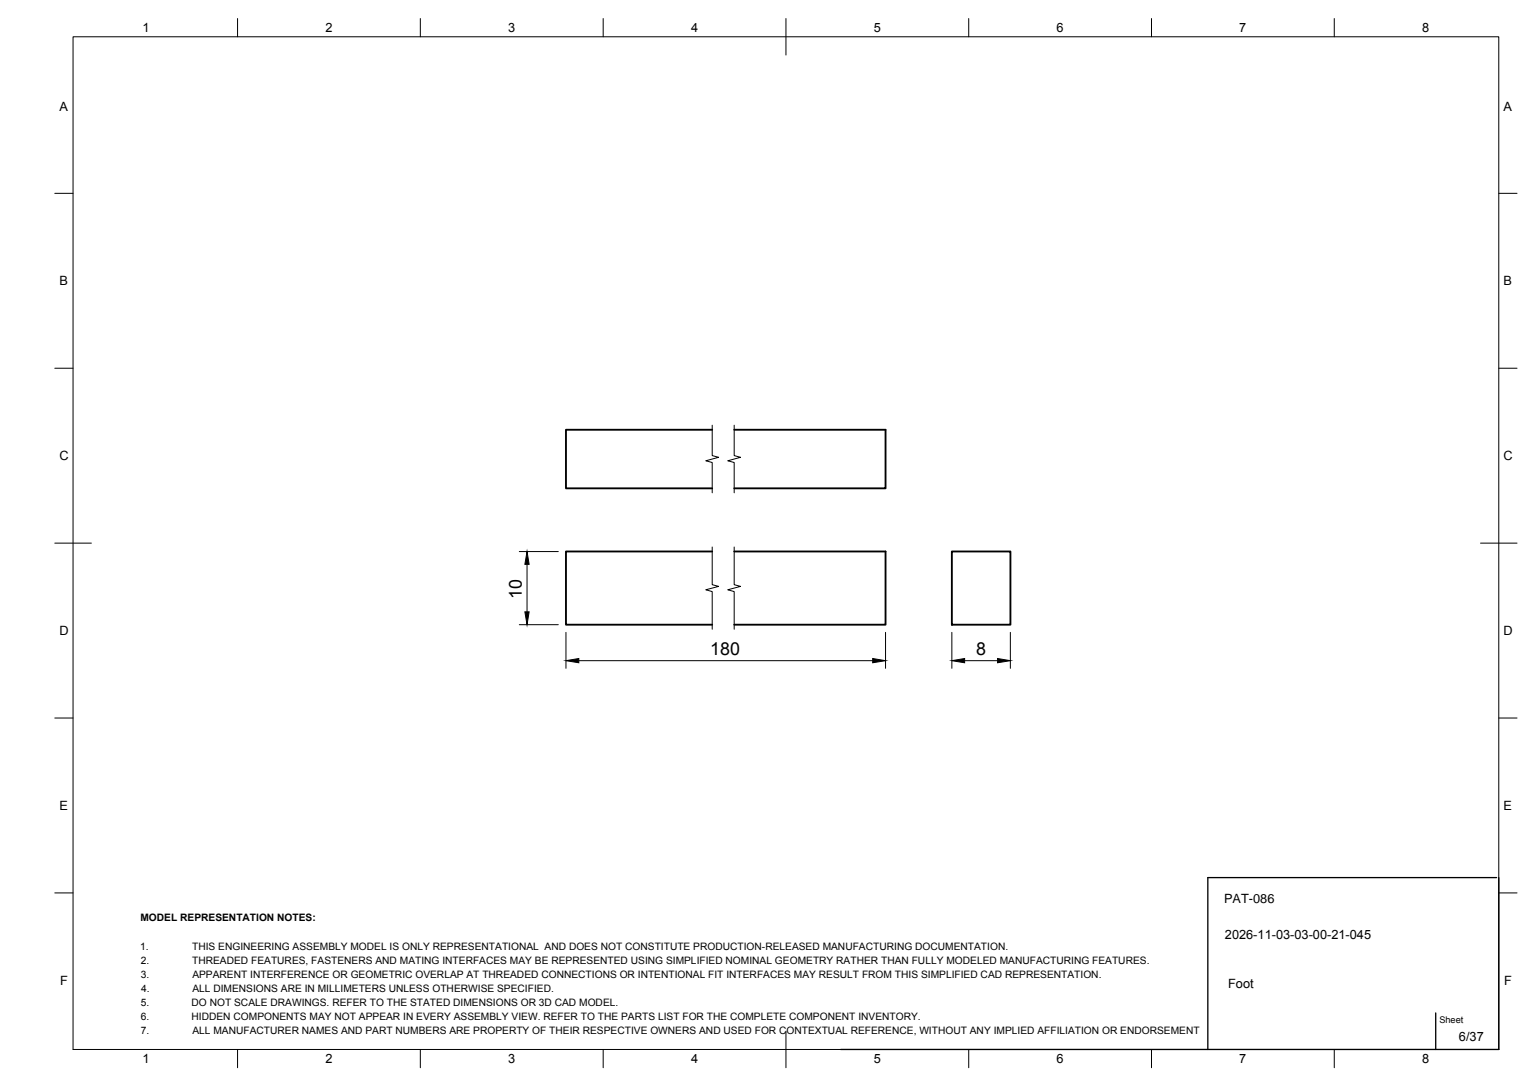
ISO-10303-21;
HEADER;
/* Generated by software containing ST-Developer
 * from STEP Tools, Inc. (www.steptools.com) 
 */

FILE_DESCRIPTION(
/* description */ ('Ratchet and pawl hand winch drum'),
/* implementation_level */ '2;1');

FILE_NAME(
/* name */ 'Foot.step',
/* time_stamp */ '2026-10-27T12:42:58-07:00',
/* author */ (''),
/* organization */ (''),
/* preprocessor_version */ 'ST-DEVELOPER v20.2',
/* originating_system */ 'Autodesk Translation Framework v15.17.0.0',
/* authorisation */ '');

FILE_SCHEMA (('AUTOMOTIVE_DESIGN { 1 0 10303 214 3 1 1 }'));
ENDSEC;

DATA;
#10=MECHANICAL_DESIGN_GEOMETRIC_PRESENTATION_REPRESENTATION('',(#390),#11801);
#322=SHAPE_REPRESENTATION_RELATIONSHIP('SRR','None',#11948,#356);
#356=ADVANCED_BREP_SHAPE_REPRESENTATION('',(#425),#11765);
#390=STYLED_ITEM('',(#12227),#425);
#425=MANIFOLD_SOLID_BREP('Body1',#6267);
#607=PLANE('',#6719);
#608=PLANE('',#6720);
#609=PLANE('',#6721);
#610=PLANE('',#6722);
#611=PLANE('',#6723);
#612=PLANE('',#6724);
#856=FACE_OUTER_BOUND('',#1232,.T.);
#857=FACE_OUTER_BOUND('',#1233,.T.);
#858=FACE_OUTER_BOUND('',#1234,.T.);
#859=FACE_OUTER_BOUND('',#1235,.T.);
#860=FACE_OUTER_BOUND('',#1236,.T.);
#861=FACE_OUTER_BOUND('',#1237,.T.);
#1232=EDGE_LOOP('',(#4331,#4332,#4333,#4334));
#1233=EDGE_LOOP('',(#4335,#4336,#4337,#4338));
#1234=EDGE_LOOP('',(#4339,#4340,#4341,#4342));
#1235=EDGE_LOOP('',(#4343,#4344,#4345,#4346));
#1236=EDGE_LOOP('',(#4347,#4348,#4349,#4350));
#1237=EDGE_LOOP('',(#4351,#4352,#4353,#4354));
#1719=LINE('',#9320,#2230);
#1720=LINE('',#9322,#2231);
#1721=LINE('',#9324,#2232);
#1722=LINE('',#9325,#2233);
#1723=LINE('',#9328,#2234);
#1724=LINE('',#9330,#2235);
#1725=LINE('',#9331,#2236);
#1726=LINE('',#9334,#2237);
#1727=LINE('',#9336,#2238);
#1728=LINE('',#9337,#2239);
#1729=LINE('',#9339,#2240);
#1730=LINE('',#9340,#2241);
#2230=VECTOR('',#7462,1.);
#2231=VECTOR('',#7463,1.);
#2232=VECTOR('',#7464,1.);
#2233=VECTOR('',#7465,1.);
#2234=VECTOR('',#7468,1.);
#2235=VECTOR('',#7469,1.);
#2236=VECTOR('',#7470,1.);
#2237=VECTOR('',#7473,1.);
#2238=VECTOR('',#7474,1.);
#2239=VECTOR('',#7475,1.);
#2240=VECTOR('',#7478,1.);
#2241=VECTOR('',#7479,1.);
#2970=VERTEX_POINT('',#9318);
#2971=VERTEX_POINT('',#9319);
#2972=VERTEX_POINT('',#9321);
#2973=VERTEX_POINT('',#9323);
#2974=VERTEX_POINT('',#9327);
#2975=VERTEX_POINT('',#9329);
#2976=VERTEX_POINT('',#9333);
#2977=VERTEX_POINT('',#9335);
#3509=EDGE_CURVE('',#2970,#2971,#1719,.T.);
#3510=EDGE_CURVE('',#2971,#2972,#1720,.T.);
#3511=EDGE_CURVE('',#2973,#2972,#1721,.T.);
#3512=EDGE_CURVE('',#2970,#2973,#1722,.T.);
#3513=EDGE_CURVE('',#2974,#2970,#1723,.T.);
#3514=EDGE_CURVE('',#2975,#2973,#1724,.T.);
#3515=EDGE_CURVE('',#2974,#2975,#1725,.T.);
#3516=EDGE_CURVE('',#2976,#2974,#1726,.T.);
#3517=EDGE_CURVE('',#2977,#2975,#1727,.T.);
#3518=EDGE_CURVE('',#2976,#2977,#1728,.T.);
#3519=EDGE_CURVE('',#2971,#2976,#1729,.T.);
#3520=EDGE_CURVE('',#2972,#2977,#1730,.T.);
#4331=ORIENTED_EDGE('',*,*,#3509,.T.);
#4332=ORIENTED_EDGE('',*,*,#3510,.T.);
#4333=ORIENTED_EDGE('',*,*,#3511,.F.);
#4334=ORIENTED_EDGE('',*,*,#3512,.F.);
#4335=ORIENTED_EDGE('',*,*,#3513,.T.);
#4336=ORIENTED_EDGE('',*,*,#3512,.T.);
#4337=ORIENTED_EDGE('',*,*,#3514,.F.);
#4338=ORIENTED_EDGE('',*,*,#3515,.F.);
#4339=ORIENTED_EDGE('',*,*,#3516,.T.);
#4340=ORIENTED_EDGE('',*,*,#3515,.T.);
#4341=ORIENTED_EDGE('',*,*,#3517,.F.);
#4342=ORIENTED_EDGE('',*,*,#3518,.F.);
#4343=ORIENTED_EDGE('',*,*,#3519,.T.);
#4344=ORIENTED_EDGE('',*,*,#3518,.T.);
#4345=ORIENTED_EDGE('',*,*,#3520,.F.);
#4346=ORIENTED_EDGE('',*,*,#3510,.F.);
#4347=ORIENTED_EDGE('',*,*,#3520,.T.);
#4348=ORIENTED_EDGE('',*,*,#3517,.T.);
#4349=ORIENTED_EDGE('',*,*,#3514,.T.);
#4350=ORIENTED_EDGE('',*,*,#3511,.T.);
#4351=ORIENTED_EDGE('',*,*,#3519,.F.);
#4352=ORIENTED_EDGE('',*,*,#3509,.F.);
#4353=ORIENTED_EDGE('',*,*,#3513,.F.);
#4354=ORIENTED_EDGE('',*,*,#3516,.F.);
#5926=ADVANCED_FACE('',(#856),#607,.T.);
#5927=ADVANCED_FACE('',(#857),#608,.T.);
#5928=ADVANCED_FACE('',(#858),#609,.T.);
#5929=ADVANCED_FACE('',(#859),#610,.T.);
#5930=ADVANCED_FACE('',(#860),#611,.T.);
#5931=ADVANCED_FACE('',(#861),#612,.F.);
#6267=CLOSED_SHELL('',(#5926,#5927,#5928,#5929,#5930,#5931));
#6718=AXIS2_PLACEMENT_3D('',#9316,#7458,#7459);
#6719=AXIS2_PLACEMENT_3D('',#9317,#7460,#7461);
#6720=AXIS2_PLACEMENT_3D('',#9326,#7466,#7467);
#6721=AXIS2_PLACEMENT_3D('',#9332,#7471,#7472);
#6722=AXIS2_PLACEMENT_3D('',#9338,#7476,#7477);
#6723=AXIS2_PLACEMENT_3D('',#9341,#7480,#7481);
#6724=AXIS2_PLACEMENT_3D('',#9342,#7482,#7483);
#7458=DIRECTION('axis',(0.,0.,1.));
#7459=DIRECTION('refdir',(1.,0.,0.));
#7460=DIRECTION('center_axis',(0.,1.,0.));
#7461=DIRECTION('ref_axis',(-1.,0.,0.));
#7462=DIRECTION('',(-1.,0.,0.));
#7463=DIRECTION('',(0.,0.,1.));
#7464=DIRECTION('',(-1.,0.,0.));
#7465=DIRECTION('',(0.,0.,1.));
#7466=DIRECTION('center_axis',(1.,0.,0.));
#7467=DIRECTION('ref_axis',(0.,1.,0.));
#7468=DIRECTION('',(0.,1.,0.));
#7469=DIRECTION('',(0.,1.,0.));
#7470=DIRECTION('',(0.,0.,1.));
#7471=DIRECTION('center_axis',(0.,-1.,0.));
#7472=DIRECTION('ref_axis',(1.,0.,0.));
#7473=DIRECTION('',(1.,0.,0.));
#7474=DIRECTION('',(1.,0.,0.));
#7475=DIRECTION('',(0.,0.,1.));
#7476=DIRECTION('center_axis',(-1.,0.,0.));
#7477=DIRECTION('ref_axis',(0.,-1.,0.));
#7478=DIRECTION('',(0.,-1.,0.));
#7479=DIRECTION('',(0.,-1.,0.));
#7480=DIRECTION('center_axis',(0.,0.,1.));
#7481=DIRECTION('ref_axis',(1.,0.,0.));
#7482=DIRECTION('center_axis',(0.,0.,1.));
#7483=DIRECTION('ref_axis',(1.,0.,0.));
#9316=CARTESIAN_POINT('',(0.,0.,0.));
#9317=CARTESIAN_POINT('Origin',(10.,-7.5,-0.8));
#9318=CARTESIAN_POINT('',(10.,-7.5,-0.8));
#9319=CARTESIAN_POINT('',(-8.,-7.5,-0.8));
#9320=CARTESIAN_POINT('',(10.,-7.5,-0.8));
#9321=CARTESIAN_POINT('',(-8.,-7.5,0.));
#9322=CARTESIAN_POINT('',(-8.,-7.5,-0.8));
#9323=CARTESIAN_POINT('',(10.,-7.5,0.));
#9324=CARTESIAN_POINT('',(10.,-7.5,0.));
#9325=CARTESIAN_POINT('',(10.,-7.5,-0.8));
#9326=CARTESIAN_POINT('Origin',(10.,-8.5,-0.8));
#9327=CARTESIAN_POINT('',(10.,-8.5,-0.8));
#9328=CARTESIAN_POINT('',(10.,-8.5,-0.8));
#9329=CARTESIAN_POINT('',(10.,-8.5,0.));
#9330=CARTESIAN_POINT('',(10.,-8.5,0.));
#9331=CARTESIAN_POINT('',(10.,-8.5,-0.8));
#9332=CARTESIAN_POINT('Origin',(-8.,-8.5,-0.8));
#9333=CARTESIAN_POINT('',(-8.,-8.5,-0.8));
#9334=CARTESIAN_POINT('',(-8.,-8.5,-0.8));
#9335=CARTESIAN_POINT('',(-8.,-8.5,0.));
#9336=CARTESIAN_POINT('',(-8.,-8.5,0.));
#9337=CARTESIAN_POINT('',(-8.,-8.5,-0.8));
#9338=CARTESIAN_POINT('Origin',(-8.,-7.5,-0.8));
#9339=CARTESIAN_POINT('',(-8.,-7.5,-0.8));
#9340=CARTESIAN_POINT('',(-8.,-7.5,0.));
#9341=CARTESIAN_POINT('Origin',(1.,-8.,0.));
#9342=CARTESIAN_POINT('Origin',(1.,-8.,-0.8));
#11725=UNCERTAINTY_MEASURE_WITH_UNIT(LENGTH_MEASURE(0.001),#11802,
'DISTANCE_ACCURACY_VALUE',
'Maximum model space distance between geometric entities at asserted c
onnectivities');
#11761=UNCERTAINTY_MEASURE_WITH_UNIT(LENGTH_MEASURE(0.001),#11802,
'DISTANCE_ACCURACY_VALUE',
'Maximum model space distance between geometric entities at asserted c
onnectivities');
#11765=(
GEOMETRIC_REPRESENTATION_CONTEXT(3)
GLOBAL_UNCERTAINTY_ASSIGNED_CONTEXT((#11725))
GLOBAL_UNIT_ASSIGNED_CONTEXT((#11802,#11804,#11805))
REPRESENTATION_CONTEXT('','3D')
);
#11801=(
GEOMETRIC_REPRESENTATION_CONTEXT(3)
GLOBAL_UNCERTAINTY_ASSIGNED_CONTEXT((#11761))
GLOBAL_UNIT_ASSIGNED_CONTEXT((#11802,#11804,#11805))
REPRESENTATION_CONTEXT('','3D')
);
#11802=(
LENGTH_UNIT()
NAMED_UNIT(*)
SI_UNIT(.CENTI.,.METRE.)
);
#11804=(
NAMED_UNIT(*)
PLANE_ANGLE_UNIT()
SI_UNIT($,.RADIAN.)
);
#11805=(
NAMED_UNIT(*)
SI_UNIT($,.STERADIAN.)
SOLID_ANGLE_UNIT()
);
#11809=SHAPE_DEFINITION_REPRESENTATION(#11848,#11948);
#11848=PRODUCT_DEFINITION_SHAPE('',$,#11988);
#11948=SHAPE_REPRESENTATION('',(#6718),#11765);
#11984=PRODUCT_DEFINITION_CONTEXT('part definition',#12103,'design');
#11988=PRODUCT_DEFINITION('Foot','Foot',#12027,#11984);
#12027=PRODUCT_DEFINITION_FORMATION('',$,#12108);
#12103=APPLICATION_CONTEXT(
'Core Data for Automotive Mechanical Design Process');
#12104=PRODUCT_CONTEXT('part definition',#12103,'mechanical');
#12108=PRODUCT('Foot','Foot','Foot',(#12104));
#12221=COLOUR_RGB('Off White',0.89,0.88,0.83);
#12222=FILL_AREA_STYLE_COLOUR('',#12221);
#12223=FILL_AREA_STYLE('',(#12222));
#12224=SURFACE_STYLE_FILL_AREA(#12223);
#12225=SURFACE_SIDE_STYLE('',(#12224));
#12226=SURFACE_STYLE_USAGE(.BOTH.,#12225);
#12227=PRESENTATION_STYLE_ASSIGNMENT((#12226));
ENDSEC;
END-ISO-10303-21;
